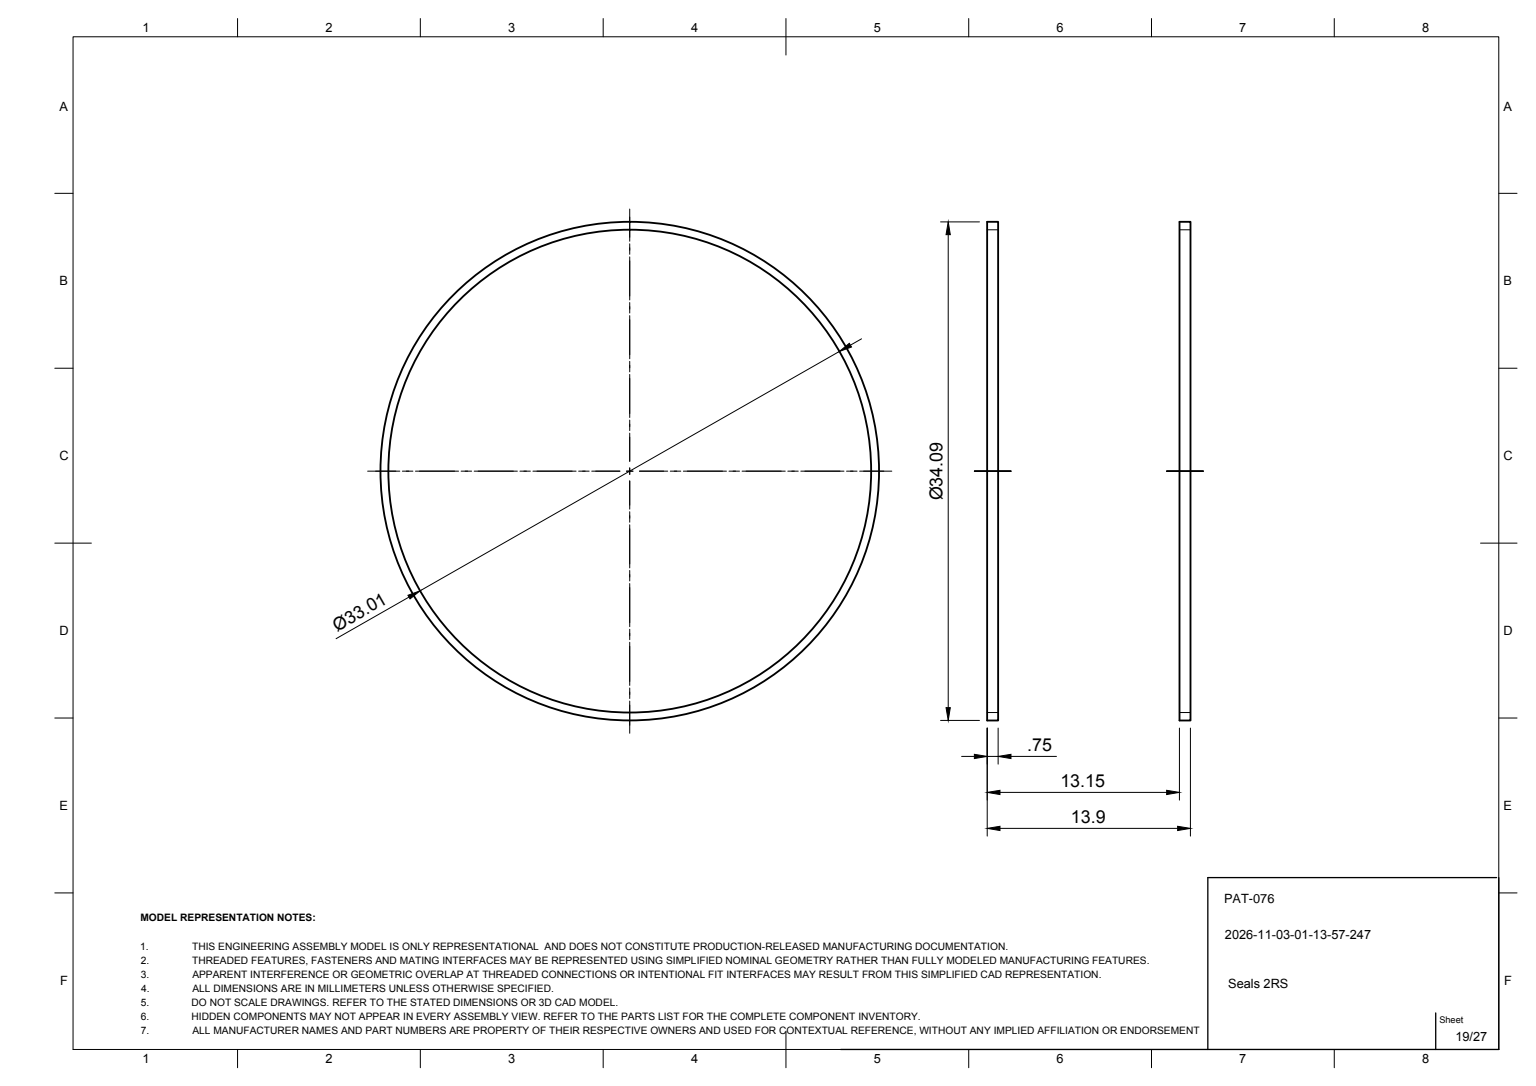
ISO-10303-21;
HEADER;
/* Generated by software containing ST-Developer
 * from STEP Tools, Inc. (www.steptools.com) 
 */

FILE_DESCRIPTION(
/* description */ ('Overhung pulley bearing cartridge'),
/* implementation_level */ '2;1');

FILE_NAME(
/* name */ 'Seals 2RS.step',
/* time_stamp */ '2026-10-28T03:22:33-07:00',
/* author */ (''),
/* organization */ (''),
/* preprocessor_version */ 'ST-DEVELOPER v20.2',
/* originating_system */ 'Autodesk Translation Framework v15.17.0.0',
/* authorisation */ '');

FILE_SCHEMA (('AUTOMOTIVE_DESIGN { 1 0 10303 214 3 1 1 }'));
ENDSEC;

DATA;
#10=MECHANICAL_DESIGN_GEOMETRIC_PRESENTATION_REPRESENTATION('',(#302,#303),#10963);
#251=SHAPE_REPRESENTATION_RELATIONSHIP('SRR','None',#11072,#273);
#273=ADVANCED_BREP_SHAPE_REPRESENTATION('',(#332,#333),#10952);
#302=STYLED_ITEM('',(#11253),#332);
#303=STYLED_ITEM('',(#11253),#333);
#332=MANIFOLD_SOLID_BREP('Body1',#5669);
#333=MANIFOLD_SOLID_BREP('Body2',#5670);
#401=FACE_BOUND('',#1104,.T.);
#402=FACE_BOUND('',#1107,.T.);
#403=FACE_BOUND('',#1110,.T.);
#404=FACE_BOUND('',#1113,.T.);
#504=PLANE('',#6224);
#505=PLANE('',#6229);
#506=PLANE('',#6232);
#507=PLANE('',#6237);
#714=FACE_OUTER_BOUND('',#1103,.T.);
#715=FACE_OUTER_BOUND('',#1105,.T.);
#716=FACE_OUTER_BOUND('',#1106,.T.);
#717=FACE_OUTER_BOUND('',#1108,.T.);
#718=FACE_OUTER_BOUND('',#1109,.T.);
#719=FACE_OUTER_BOUND('',#1111,.T.);
#720=FACE_OUTER_BOUND('',#1112,.T.);
#721=FACE_OUTER_BOUND('',#1114,.T.);
#1103=EDGE_LOOP('',(#4223));
#1104=EDGE_LOOP('',(#4224));
#1105=EDGE_LOOP('',(#4225,#4226,#4227,#4228));
#1106=EDGE_LOOP('',(#4229));
#1107=EDGE_LOOP('',(#4230));
#1108=EDGE_LOOP('',(#4231,#4232,#4233,#4234));
#1109=EDGE_LOOP('',(#4235));
#1110=EDGE_LOOP('',(#4236));
#1111=EDGE_LOOP('',(#4237,#4238,#4239,#4240));
#1112=EDGE_LOOP('',(#4241));
#1113=EDGE_LOOP('',(#4242));
#1114=EDGE_LOOP('',(#4243,#4244,#4245,#4246));
#1449=LINE('',#9538,#1791);
#1450=LINE('',#9543,#1792);
#1451=LINE('',#9552,#1793);
#1452=LINE('',#9557,#1794);
#1791=VECTOR('',#7417,1.70469);
#1792=VECTOR('',#7424,1.65031);
#1793=VECTOR('',#7435,1.70469);
#1794=VECTOR('',#7442,1.65031);
#2158=CIRCLE('',#6225,1.70469);
#2159=CIRCLE('',#6226,1.65031);
#2160=CIRCLE('',#6228,1.70469);
#2161=CIRCLE('',#6230,1.65031);
#2162=CIRCLE('',#6233,1.70469);
#2163=CIRCLE('',#6234,1.65031);
#2164=CIRCLE('',#6236,1.70469);
#2165=CIRCLE('',#6238,1.65031);
#2581=VERTEX_POINT('',#9531);
#2582=VERTEX_POINT('',#9533);
#2583=VERTEX_POINT('',#9536);
#2584=VERTEX_POINT('',#9540);
#2585=VERTEX_POINT('',#9545);
#2586=VERTEX_POINT('',#9547);
#2587=VERTEX_POINT('',#9550);
#2588=VERTEX_POINT('',#9554);
#3181=EDGE_CURVE('',#2581,#2581,#2158,.T.);
#3182=EDGE_CURVE('',#2582,#2582,#2159,.T.);
#3183=EDGE_CURVE('',#2583,#2583,#2160,.T.);
#3184=EDGE_CURVE('',#2583,#2581,#1449,.T.);
#3185=EDGE_CURVE('',#2584,#2584,#2161,.T.);
#3186=EDGE_CURVE('',#2584,#2582,#1450,.T.);
#3187=EDGE_CURVE('',#2585,#2585,#2162,.T.);
#3188=EDGE_CURVE('',#2586,#2586,#2163,.T.);
#3189=EDGE_CURVE('',#2587,#2587,#2164,.T.);
#3190=EDGE_CURVE('',#2587,#2585,#1451,.T.);
#3191=EDGE_CURVE('',#2588,#2588,#2165,.T.);
#3192=EDGE_CURVE('',#2588,#2586,#1452,.T.);
#4223=ORIENTED_EDGE('',*,*,#3181,.F.);
#4224=ORIENTED_EDGE('',*,*,#3182,.T.);
#4225=ORIENTED_EDGE('',*,*,#3183,.F.);
#4226=ORIENTED_EDGE('',*,*,#3184,.T.);
#4227=ORIENTED_EDGE('',*,*,#3181,.T.);
#4228=ORIENTED_EDGE('',*,*,#3184,.F.);
#4229=ORIENTED_EDGE('',*,*,#3183,.T.);
#4230=ORIENTED_EDGE('',*,*,#3185,.F.);
#4231=ORIENTED_EDGE('',*,*,#3185,.T.);
#4232=ORIENTED_EDGE('',*,*,#3186,.T.);
#4233=ORIENTED_EDGE('',*,*,#3182,.F.);
#4234=ORIENTED_EDGE('',*,*,#3186,.F.);
#4235=ORIENTED_EDGE('',*,*,#3187,.F.);
#4236=ORIENTED_EDGE('',*,*,#3188,.T.);
#4237=ORIENTED_EDGE('',*,*,#3189,.F.);
#4238=ORIENTED_EDGE('',*,*,#3190,.T.);
#4239=ORIENTED_EDGE('',*,*,#3187,.T.);
#4240=ORIENTED_EDGE('',*,*,#3190,.F.);
#4241=ORIENTED_EDGE('',*,*,#3189,.T.);
#4242=ORIENTED_EDGE('',*,*,#3191,.F.);
#4243=ORIENTED_EDGE('',*,*,#3191,.T.);
#4244=ORIENTED_EDGE('',*,*,#3192,.T.);
#4245=ORIENTED_EDGE('',*,*,#3188,.F.);
#4246=ORIENTED_EDGE('',*,*,#3192,.F.);
#5212=CYLINDRICAL_SURFACE('',#6227,1.70469);
#5213=CYLINDRICAL_SURFACE('',#6231,1.65031);
#5214=CYLINDRICAL_SURFACE('',#6235,1.70469);
#5215=CYLINDRICAL_SURFACE('',#6239,1.65031);
#5458=ADVANCED_FACE('',(#714,#401),#504,.T.);
#5459=ADVANCED_FACE('',(#715),#5212,.T.);
#5460=ADVANCED_FACE('',(#716,#402),#505,.T.);
#5461=ADVANCED_FACE('',(#717),#5213,.F.);
#5462=ADVANCED_FACE('',(#718,#403),#506,.T.);
#5463=ADVANCED_FACE('',(#719),#5214,.T.);
#5464=ADVANCED_FACE('',(#720,#404),#507,.T.);
#5465=ADVANCED_FACE('',(#721),#5215,.F.);
#5669=CLOSED_SHELL('',(#5458,#5459,#5460,#5461));
#5670=CLOSED_SHELL('',(#5462,#5463,#5464,#5465));
#6223=AXIS2_PLACEMENT_3D('',#9529,#7405,#7406);
#6224=AXIS2_PLACEMENT_3D('',#9530,#7407,#7408);
#6225=AXIS2_PLACEMENT_3D('',#9532,#7409,#7410);
#6226=AXIS2_PLACEMENT_3D('',#9534,#7411,#7412);
#6227=AXIS2_PLACEMENT_3D('',#9535,#7413,#7414);
#6228=AXIS2_PLACEMENT_3D('',#9537,#7415,#7416);
#6229=AXIS2_PLACEMENT_3D('',#9539,#7418,#7419);
#6230=AXIS2_PLACEMENT_3D('',#9541,#7420,#7421);
#6231=AXIS2_PLACEMENT_3D('',#9542,#7422,#7423);
#6232=AXIS2_PLACEMENT_3D('',#9544,#7425,#7426);
#6233=AXIS2_PLACEMENT_3D('',#9546,#7427,#7428);
#6234=AXIS2_PLACEMENT_3D('',#9548,#7429,#7430);
#6235=AXIS2_PLACEMENT_3D('',#9549,#7431,#7432);
#6236=AXIS2_PLACEMENT_3D('',#9551,#7433,#7434);
#6237=AXIS2_PLACEMENT_3D('',#9553,#7436,#7437);
#6238=AXIS2_PLACEMENT_3D('',#9555,#7438,#7439);
#6239=AXIS2_PLACEMENT_3D('',#9556,#7440,#7441);
#7405=DIRECTION('axis',(0.,0.,1.));
#7406=DIRECTION('refdir',(1.,0.,0.));
#7407=DIRECTION('center_axis',(0.,1.,0.));
#7408=DIRECTION('ref_axis',(0.,0.,1.));
#7409=DIRECTION('center_axis',(0.,-1.,0.));
#7410=DIRECTION('ref_axis',(1.,0.,0.));
#7411=DIRECTION('center_axis',(0.,-1.,0.));
#7412=DIRECTION('ref_axis',(1.,0.,0.));
#7413=DIRECTION('center_axis',(0.,-1.,0.));
#7414=DIRECTION('ref_axis',(1.,0.,0.));
#7415=DIRECTION('center_axis',(0.,-1.,0.));
#7416=DIRECTION('ref_axis',(1.,0.,0.));
#7417=DIRECTION('',(0.,1.,0.));
#7418=DIRECTION('center_axis',(0.,-1.,0.));
#7419=DIRECTION('ref_axis',(0.,0.,-1.));
#7420=DIRECTION('center_axis',(0.,-1.,0.));
#7421=DIRECTION('ref_axis',(1.,0.,0.));
#7422=DIRECTION('center_axis',(0.,-1.,0.));
#7423=DIRECTION('ref_axis',(1.,0.,0.));
#7424=DIRECTION('',(0.,1.,0.));
#7425=DIRECTION('center_axis',(0.,1.,0.));
#7426=DIRECTION('ref_axis',(0.,0.,1.));
#7427=DIRECTION('center_axis',(0.,-1.,0.));
#7428=DIRECTION('ref_axis',(1.,0.,0.));
#7429=DIRECTION('center_axis',(0.,-1.,0.));
#7430=DIRECTION('ref_axis',(1.,0.,0.));
#7431=DIRECTION('center_axis',(0.,-1.,0.));
#7432=DIRECTION('ref_axis',(1.,0.,0.));
#7433=DIRECTION('center_axis',(0.,-1.,0.));
#7434=DIRECTION('ref_axis',(1.,0.,0.));
#7435=DIRECTION('',(0.,1.,0.));
#7436=DIRECTION('center_axis',(0.,-1.,0.));
#7437=DIRECTION('ref_axis',(0.,0.,-1.));
#7438=DIRECTION('center_axis',(0.,-1.,0.));
#7439=DIRECTION('ref_axis',(1.,0.,0.));
#7440=DIRECTION('center_axis',(0.,-1.,0.));
#7441=DIRECTION('ref_axis',(1.,0.,0.));
#7442=DIRECTION('',(0.,1.,0.));
#9529=CARTESIAN_POINT('',(0.,0.,0.));
#9530=CARTESIAN_POINT('Origin',(1.70469,0.695,0.));
#9531=CARTESIAN_POINT('',(-1.70469,0.695,-2.0876431520385E-16));
#9532=CARTESIAN_POINT('Origin',(0.,0.695,0.));
#9533=CARTESIAN_POINT('',(-1.65031,0.695,-2.02104685910087E-16));
#9534=CARTESIAN_POINT('Origin',(0.,0.695,0.));
#9535=CARTESIAN_POINT('Origin',(0.,0.6575,0.));
#9536=CARTESIAN_POINT('',(-1.70469,0.62,-2.0876431520385E-16));
#9537=CARTESIAN_POINT('Origin',(0.,0.62,0.));
#9538=CARTESIAN_POINT('',(-1.70469,0.6575,-2.0876431520385E-16));
#9539=CARTESIAN_POINT('Origin',(1.65031,0.62,0.));
#9540=CARTESIAN_POINT('',(-1.65031,0.62,-2.02104685910087E-16));
#9541=CARTESIAN_POINT('Origin',(0.,0.62,0.));
#9542=CARTESIAN_POINT('Origin',(0.,0.6575,0.));
#9543=CARTESIAN_POINT('',(-1.65031,0.6575,-2.02104685910087E-16));
#9544=CARTESIAN_POINT('Origin',(1.70469,-0.62,0.));
#9545=CARTESIAN_POINT('',(-1.70469,-0.62,-2.0876431520385E-16));
#9546=CARTESIAN_POINT('Origin',(0.,-0.62,0.));
#9547=CARTESIAN_POINT('',(-1.65031,-0.62,-2.02104685910087E-16));
#9548=CARTESIAN_POINT('Origin',(0.,-0.62,0.));
#9549=CARTESIAN_POINT('Origin',(0.,-0.6575,0.));
#9550=CARTESIAN_POINT('',(-1.70469,-0.695,-2.0876431520385E-16));
#9551=CARTESIAN_POINT('Origin',(0.,-0.695,0.));
#9552=CARTESIAN_POINT('',(-1.70469,-0.6575,-2.0876431520385E-16));
#9553=CARTESIAN_POINT('Origin',(1.65031,-0.695,0.));
#9554=CARTESIAN_POINT('',(-1.65031,-0.695,-2.02104685910087E-16));
#9555=CARTESIAN_POINT('Origin',(0.,-0.695,0.));
#9556=CARTESIAN_POINT('Origin',(0.,-0.6575,0.));
#9557=CARTESIAN_POINT('',(-1.65031,-0.6575,-2.02104685910087E-16));
#10925=UNCERTAINTY_MEASURE_WITH_UNIT(LENGTH_MEASURE(0.001),#10964,
'DISTANCE_ACCURACY_VALUE',
'Maximum model space distance between geometric entities at asserted c
onnectivities');
#10936=UNCERTAINTY_MEASURE_WITH_UNIT(LENGTH_MEASURE(0.001),#10964,
'DISTANCE_ACCURACY_VALUE',
'Maximum model space distance between geometric entities at asserted c
onnectivities');
#10952=(
GEOMETRIC_REPRESENTATION_CONTEXT(3)
GLOBAL_UNCERTAINTY_ASSIGNED_CONTEXT((#10925))
GLOBAL_UNIT_ASSIGNED_CONTEXT((#10964,#10966,#10967))
REPRESENTATION_CONTEXT('','3D')
);
#10963=(
GEOMETRIC_REPRESENTATION_CONTEXT(3)
GLOBAL_UNCERTAINTY_ASSIGNED_CONTEXT((#10936))
GLOBAL_UNIT_ASSIGNED_CONTEXT((#10964,#10966,#10967))
REPRESENTATION_CONTEXT('','3D')
);
#10964=(
LENGTH_UNIT()
NAMED_UNIT(*)
SI_UNIT(.CENTI.,.METRE.)
);
#10966=(
NAMED_UNIT(*)
PLANE_ANGLE_UNIT()
SI_UNIT($,.RADIAN.)
);
#10967=(
NAMED_UNIT(*)
SI_UNIT($,.STERADIAN.)
SOLID_ANGLE_UNIT()
);
#10983=SHAPE_DEFINITION_REPRESENTATION(#11009,#11072);
#11009=PRODUCT_DEFINITION_SHAPE('',$,#11099);
#11072=SHAPE_REPRESENTATION('',(#6223),#10952);
#11083=PRODUCT_DEFINITION_CONTEXT('part definition',#11163,'design');
#11099=PRODUCT_DEFINITION('Seals 2RS','Seals 2RS',#11125,#11083);
#11125=PRODUCT_DEFINITION_FORMATION('',$,#11180);
#11163=APPLICATION_CONTEXT(
'Core Data for Automotive Mechanical Design Process');
#11164=PRODUCT_CONTEXT('part definition',#11163,'mechanical');
#11180=PRODUCT('Seals 2RS','Seals 2RS','Seals 2RS',(#11164));
#11247=COLOUR_RGB('Grey',0.48,0.52,0.57);
#11248=FILL_AREA_STYLE_COLOUR('',#11247);
#11249=FILL_AREA_STYLE('',(#11248));
#11250=SURFACE_STYLE_FILL_AREA(#11249);
#11251=SURFACE_SIDE_STYLE('',(#11250));
#11252=SURFACE_STYLE_USAGE(.BOTH.,#11251);
#11253=PRESENTATION_STYLE_ASSIGNMENT((#11252));
ENDSEC;
END-ISO-10303-21;
